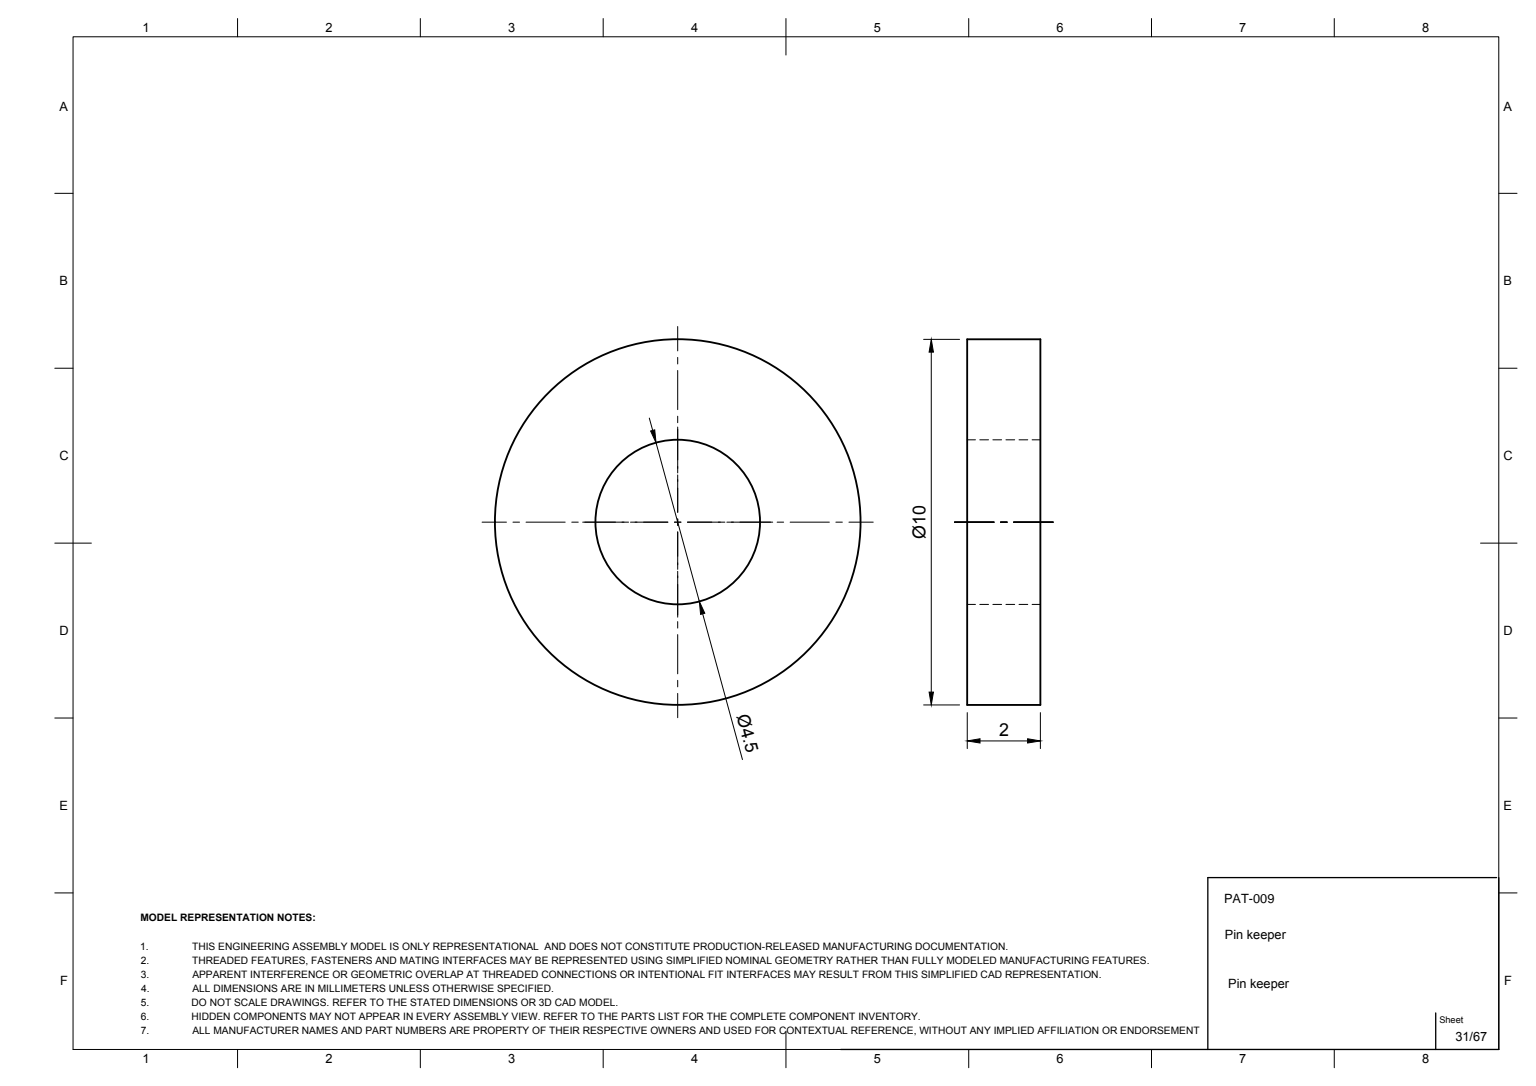
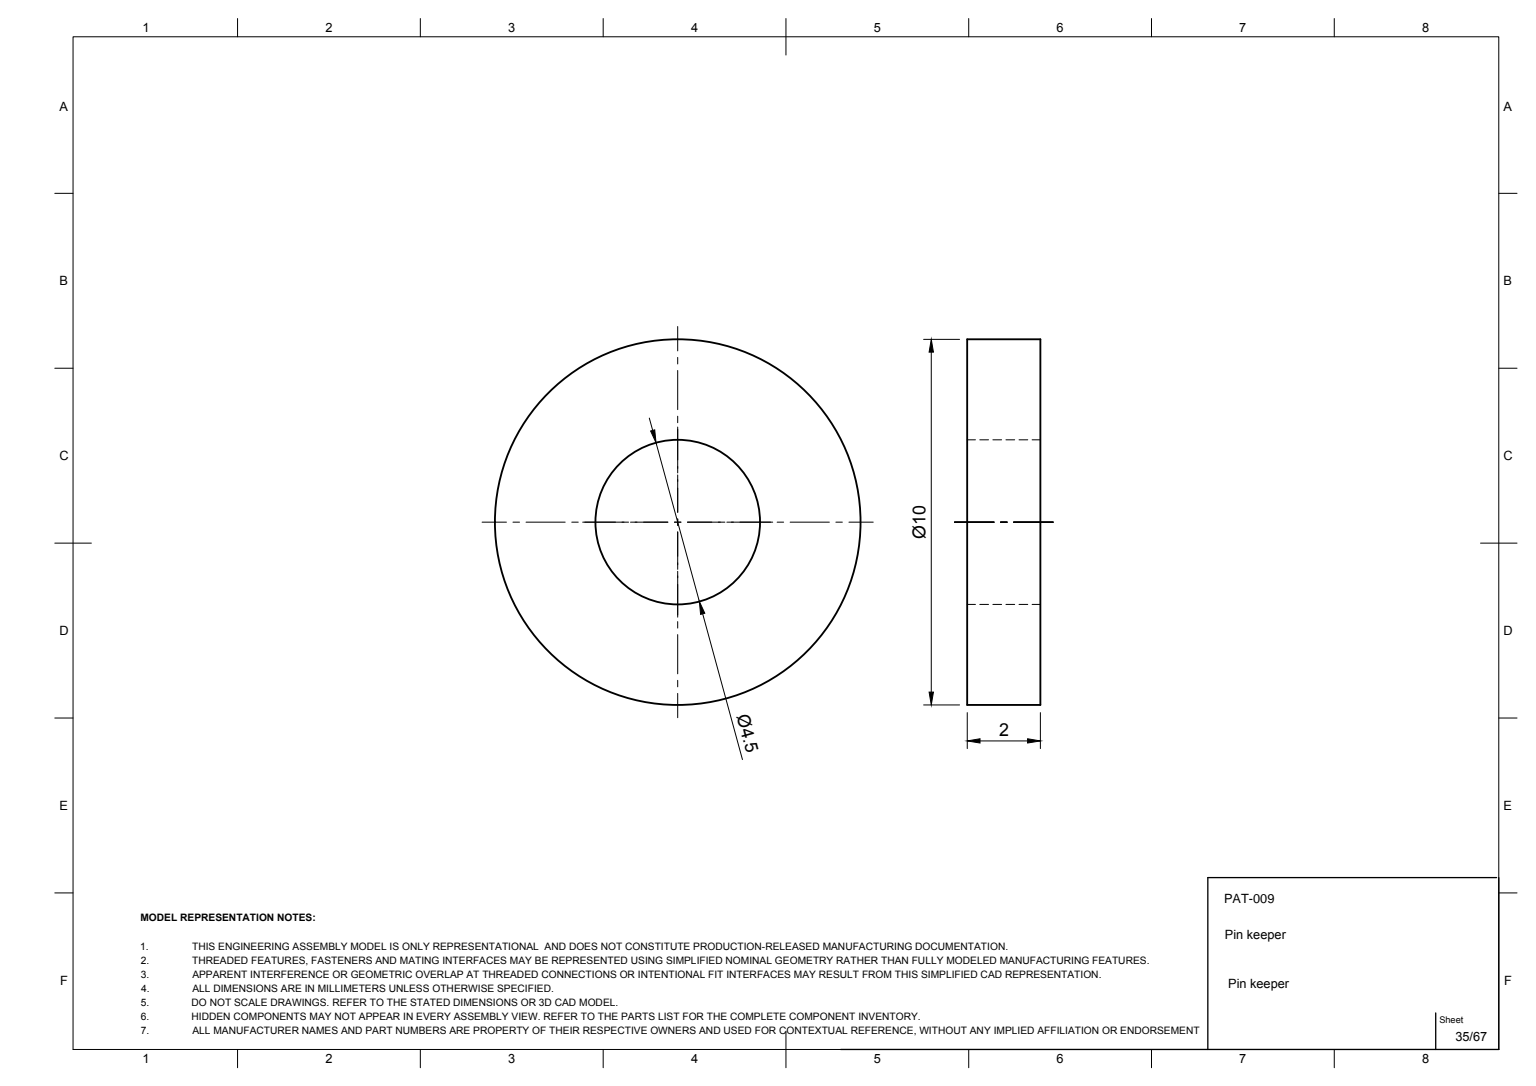
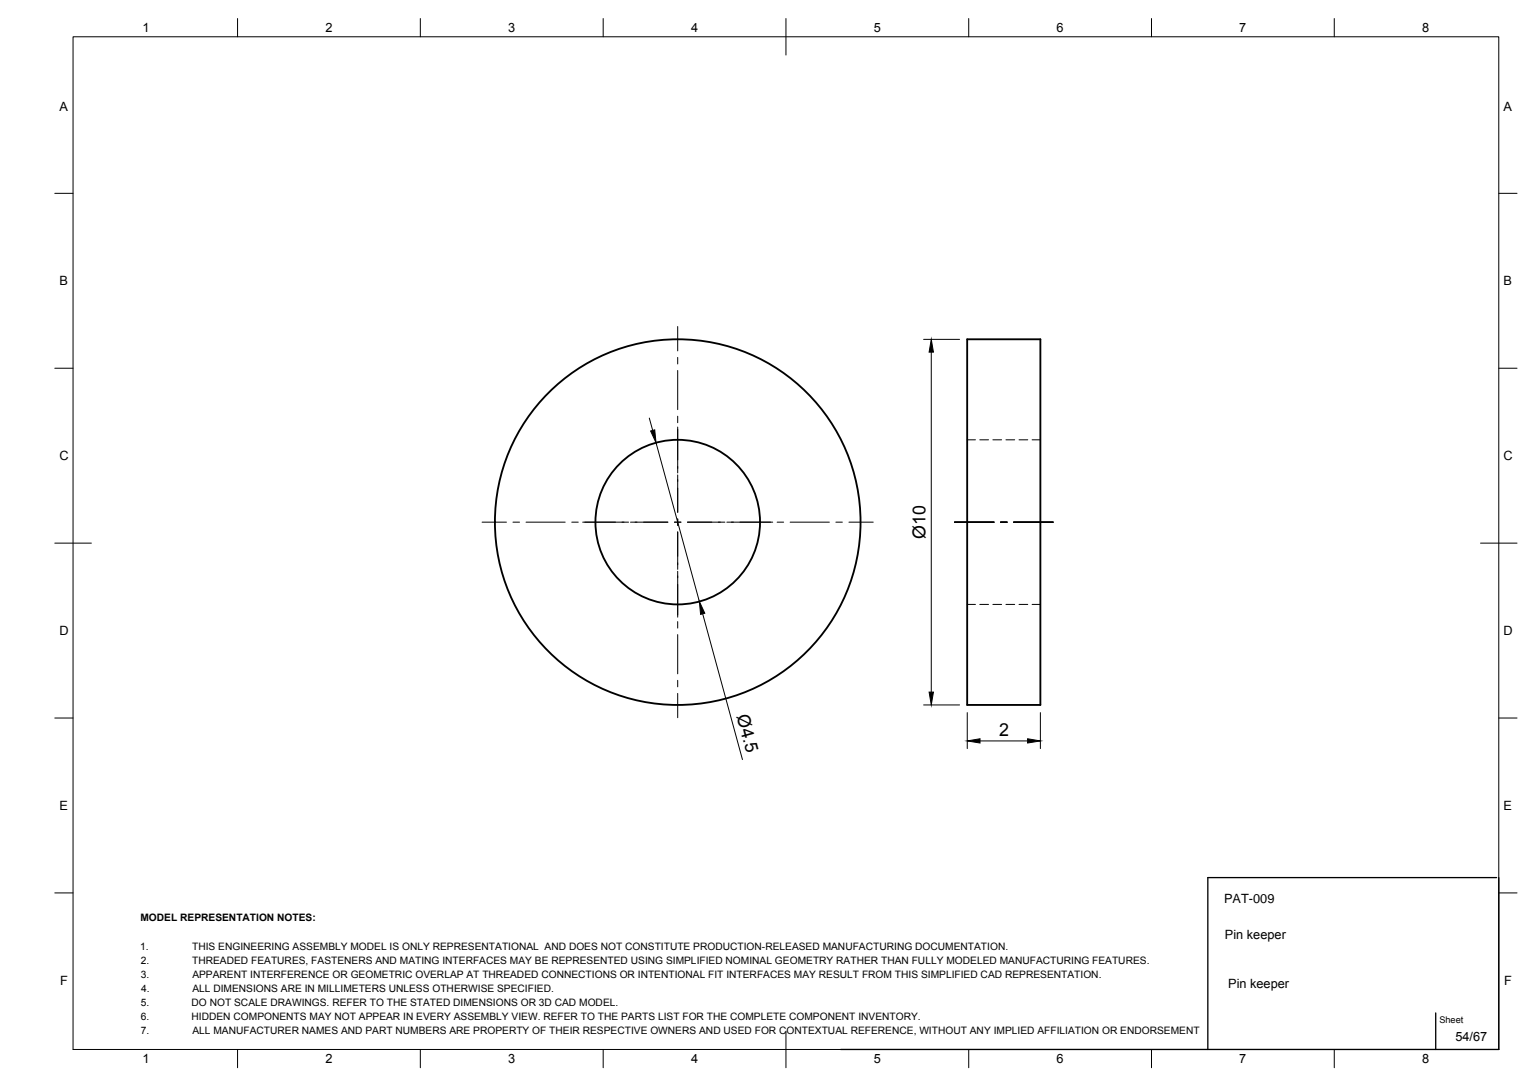
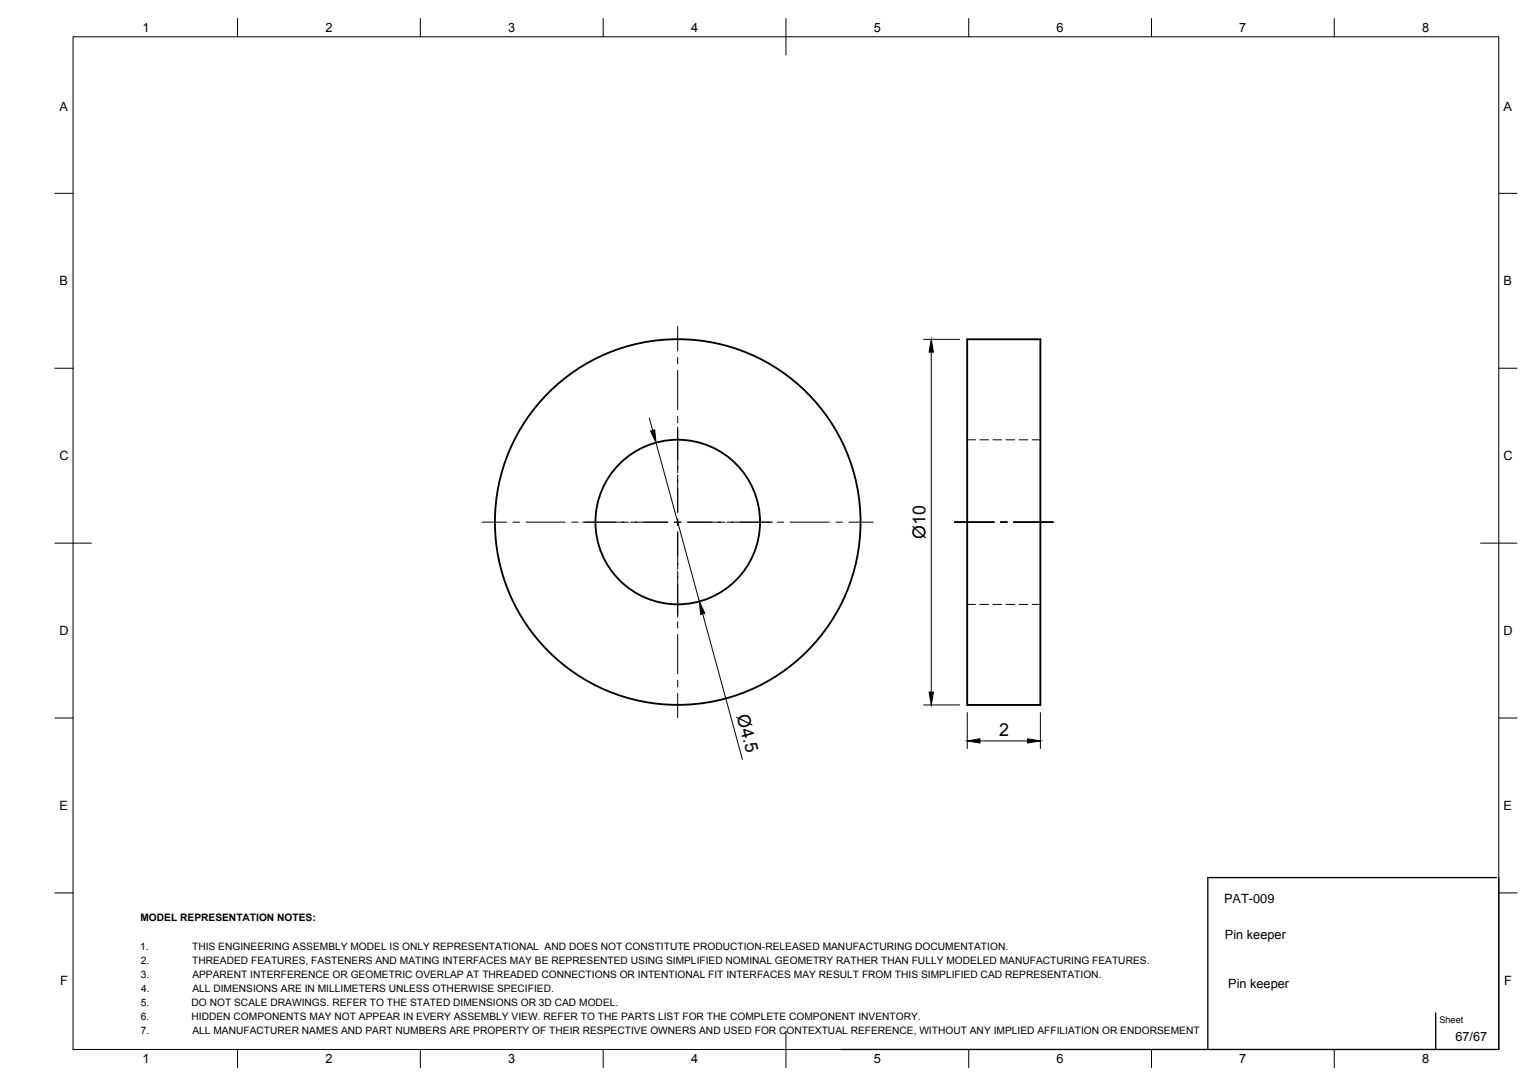
ISO-10303-21;
HEADER;
/* Generated by software containing ST-Developer
 * from STEP Tools, Inc. (www.steptools.com) 
 */

FILE_DESCRIPTION(
/* description */ ('Bell-crank linkage with push rods'),
/* implementation_level */ '2;1');

FILE_NAME(
/* name */ 'Pin keeper.step',
/* time_stamp */ '2026-10-28T03:25:15-07:00',
/* author */ (''),
/* organization */ (''),
/* preprocessor_version */ 'ST-DEVELOPER v20.2',
/* originating_system */ 'Autodesk Translation Framework v15.17.0.0',
/* authorisation */ '');

FILE_SCHEMA (('AUTOMOTIVE_DESIGN { 1 0 10303 214 3 1 1 }'));
ENDSEC;

DATA;
#10=MECHANICAL_DESIGN_GEOMETRIC_PRESENTATION_REPRESENTATION('',(#636),#16678);
#520=SHAPE_REPRESENTATION_RELATIONSHIP('SRR','None',#16938,#574);
#574=ADVANCED_BREP_SHAPE_REPRESENTATION('',(#697),#16643);
#636=STYLED_ITEM('',(#17291),#697);
#697=MANIFOLD_SOLID_BREP('Body1',#8827);
#845=FACE_BOUND('',#2176,.T.);
#846=FACE_BOUND('',#2178,.T.);
#1110=PLANE('',#10068);
#1111=PLANE('',#10069);
#1531=FACE_OUTER_BOUND('',#2173,.T.);
#1532=FACE_OUTER_BOUND('',#2174,.T.);
#1533=FACE_OUTER_BOUND('',#2175,.T.);
#1534=FACE_OUTER_BOUND('',#2177,.T.);
#2173=EDGE_LOOP('',(#7153,#7154,#7155,#7156));
#2174=EDGE_LOOP('',(#7157,#7158,#7159,#7160));
#2175=EDGE_LOOP('',(#7161));
#2176=EDGE_LOOP('',(#7162));
#2177=EDGE_LOOP('',(#7163));
#2178=EDGE_LOOP('',(#7164));
#2824=LINE('',#15428,#3373);
#2825=LINE('',#15434,#3374);
#3373=VECTOR('',#12142,0.225);
#3374=VECTOR('',#12149,0.5);
#3920=CIRCLE('',#10063,0.225);
#3921=CIRCLE('',#10064,0.225);
#3922=CIRCLE('',#10066,0.5);
#3923=CIRCLE('',#10067,0.5);
#4531=VERTEX_POINT('',#15425);
#4532=VERTEX_POINT('',#15427);
#4533=VERTEX_POINT('',#15431);
#4534=VERTEX_POINT('',#15433);
#5454=EDGE_CURVE('',#4531,#4531,#3920,.T.);
#5455=EDGE_CURVE('',#4531,#4532,#2824,.T.);
#5456=EDGE_CURVE('',#4532,#4532,#3921,.T.);
#5457=EDGE_CURVE('',#4533,#4533,#3922,.T.);
#5458=EDGE_CURVE('',#4533,#4534,#2825,.T.);
#5459=EDGE_CURVE('',#4534,#4534,#3923,.T.);
#7153=ORIENTED_EDGE('',*,*,#5454,.F.);
#7154=ORIENTED_EDGE('',*,*,#5455,.T.);
#7155=ORIENTED_EDGE('',*,*,#5456,.T.);
#7156=ORIENTED_EDGE('',*,*,#5455,.F.);
#7157=ORIENTED_EDGE('',*,*,#5457,.F.);
#7158=ORIENTED_EDGE('',*,*,#5458,.T.);
#7159=ORIENTED_EDGE('',*,*,#5459,.T.);
#7160=ORIENTED_EDGE('',*,*,#5458,.F.);
#7161=ORIENTED_EDGE('',*,*,#5457,.T.);
#7162=ORIENTED_EDGE('',*,*,#5454,.T.);
#7163=ORIENTED_EDGE('',*,*,#5459,.F.);
#7164=ORIENTED_EDGE('',*,*,#5456,.F.);
#8179=CYLINDRICAL_SURFACE('',#10062,0.225);
#8180=CYLINDRICAL_SURFACE('',#10065,0.5);
#8556=ADVANCED_FACE('',(#1531),#8179,.F.);
#8557=ADVANCED_FACE('',(#1532),#8180,.T.);
#8558=ADVANCED_FACE('',(#1533,#845),#1110,.T.);
#8559=ADVANCED_FACE('',(#1534,#846),#1111,.F.);
#8827=CLOSED_SHELL('',(#8556,#8557,#8558,#8559));
#10061=AXIS2_PLACEMENT_3D('',#15423,#12136,#12137);
#10062=AXIS2_PLACEMENT_3D('',#15424,#12138,#12139);
#10063=AXIS2_PLACEMENT_3D('',#15426,#12140,#12141);
#10064=AXIS2_PLACEMENT_3D('',#15429,#12143,#12144);
#10065=AXIS2_PLACEMENT_3D('',#15430,#12145,#12146);
#10066=AXIS2_PLACEMENT_3D('',#15432,#12147,#12148);
#10067=AXIS2_PLACEMENT_3D('',#15435,#12150,#12151);
#10068=AXIS2_PLACEMENT_3D('',#15436,#12152,#12153);
#10069=AXIS2_PLACEMENT_3D('',#15437,#12154,#12155);
#12136=DIRECTION('axis',(0.,0.,1.));
#12137=DIRECTION('refdir',(1.,0.,0.));
#12138=DIRECTION('center_axis',(0.,0.,1.));
#12139=DIRECTION('ref_axis',(1.,0.,0.));
#12140=DIRECTION('center_axis',(0.,0.,-1.));
#12141=DIRECTION('ref_axis',(1.,0.,0.));
#12142=DIRECTION('',(0.,0.,-1.));
#12143=DIRECTION('center_axis',(0.,0.,-1.));
#12144=DIRECTION('ref_axis',(1.,0.,0.));
#12145=DIRECTION('center_axis',(0.,0.,1.));
#12146=DIRECTION('ref_axis',(1.,0.,0.));
#12147=DIRECTION('center_axis',(0.,0.,1.));
#12148=DIRECTION('ref_axis',(1.,0.,0.));
#12149=DIRECTION('',(0.,0.,-1.));
#12150=DIRECTION('center_axis',(0.,0.,1.));
#12151=DIRECTION('ref_axis',(1.,0.,0.));
#12152=DIRECTION('center_axis',(0.,0.,1.));
#12153=DIRECTION('ref_axis',(1.,0.,0.));
#12154=DIRECTION('center_axis',(0.,0.,1.));
#12155=DIRECTION('ref_axis',(1.,0.,0.));
#15423=CARTESIAN_POINT('',(0.,0.,0.));
#15424=CARTESIAN_POINT('Origin',(0.,2.,10.1));
#15425=CARTESIAN_POINT('',(-0.225,2.,10.3));
#15426=CARTESIAN_POINT('Origin',(0.,2.,10.3));
#15427=CARTESIAN_POINT('',(-0.225,2.,10.1));
#15428=CARTESIAN_POINT('',(-0.225,2.,10.1));
#15429=CARTESIAN_POINT('Origin',(0.,2.,10.1));
#15430=CARTESIAN_POINT('Origin',(0.,2.,10.1));
#15431=CARTESIAN_POINT('',(-0.5,2.,10.3));
#15432=CARTESIAN_POINT('Origin',(0.,2.,10.3));
#15433=CARTESIAN_POINT('',(-0.5,2.,10.1));
#15434=CARTESIAN_POINT('',(-0.5,2.,10.1));
#15435=CARTESIAN_POINT('Origin',(0.,2.,10.1));
#15436=CARTESIAN_POINT('Origin',(0.,2.,10.3));
#15437=CARTESIAN_POINT('Origin',(0.,2.,10.1));
#16579=UNCERTAINTY_MEASURE_WITH_UNIT(LENGTH_MEASURE(0.001),#16679,
'DISTANCE_ACCURACY_VALUE',
'Maximum model space distance between geometric entities at asserted c
onnectivities');
#16614=UNCERTAINTY_MEASURE_WITH_UNIT(LENGTH_MEASURE(0.001),#16679,
'DISTANCE_ACCURACY_VALUE',
'Maximum model space distance between geometric entities at asserted c
onnectivities');
#16643=(
GEOMETRIC_REPRESENTATION_CONTEXT(3)
GLOBAL_UNCERTAINTY_ASSIGNED_CONTEXT((#16579))
GLOBAL_UNIT_ASSIGNED_CONTEXT((#16679,#16681,#16682))
REPRESENTATION_CONTEXT('','3D')
);
#16678=(
GEOMETRIC_REPRESENTATION_CONTEXT(3)
GLOBAL_UNCERTAINTY_ASSIGNED_CONTEXT((#16614))
GLOBAL_UNIT_ASSIGNED_CONTEXT((#16679,#16681,#16682))
REPRESENTATION_CONTEXT('','3D')
);
#16679=(
LENGTH_UNIT()
NAMED_UNIT(*)
SI_UNIT(.CENTI.,.METRE.)
);
#16681=(
NAMED_UNIT(*)
PLANE_ANGLE_UNIT()
SI_UNIT($,.RADIAN.)
);
#16682=(
NAMED_UNIT(*)
SI_UNIT($,.STERADIAN.)
SOLID_ANGLE_UNIT()
);
#16711=SHAPE_DEFINITION_REPRESENTATION(#16779,#16938);
#16779=PRODUCT_DEFINITION_SHAPE('',$,#17002);
#16938=SHAPE_REPRESENTATION('',(#10061),#16643);
#16973=PRODUCT_DEFINITION_CONTEXT('part definition',#17164,'design');
#17002=PRODUCT_DEFINITION('Pin keeper','Pin keeper',#17065,#16973);
#17065=PRODUCT_DEFINITION_FORMATION('',$,#17194);
#17164=APPLICATION_CONTEXT(
'Core Data for Automotive Mechanical Design Process');
#17165=PRODUCT_CONTEXT('part definition',#17164,'mechanical');
#17194=PRODUCT('Pin keeper','Pin keeper','Pin keeper',(#17165));
#17285=COLOUR_RGB('Grey',0.48,0.52,0.57);
#17286=FILL_AREA_STYLE_COLOUR('',#17285);
#17287=FILL_AREA_STYLE('',(#17286));
#17288=SURFACE_STYLE_FILL_AREA(#17287);
#17289=SURFACE_SIDE_STYLE('',(#17288));
#17290=SURFACE_STYLE_USAGE(.BOTH.,#17289);
#17291=PRESENTATION_STYLE_ASSIGNMENT((#17290));
ENDSEC;
END-ISO-10303-21;
